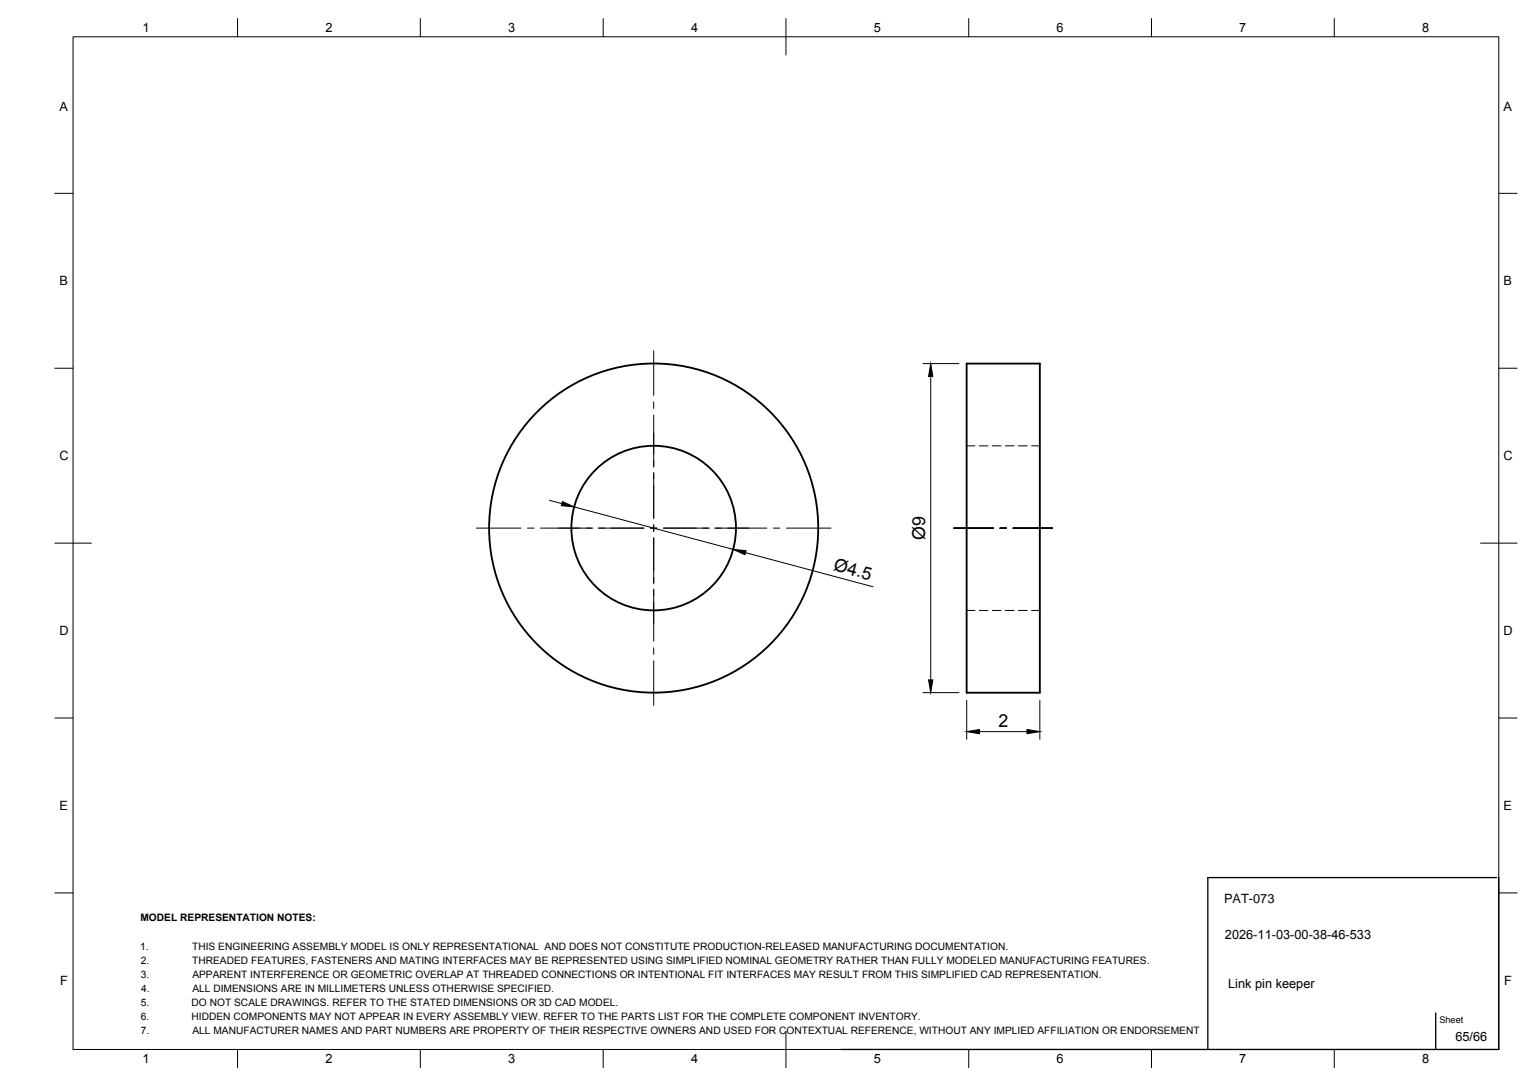
ISO-10303-21;
HEADER;
/* Generated by software containing ST-Developer
 * from STEP Tools, Inc. (www.steptools.com) 
 */

FILE_DESCRIPTION(
/* description */ ('Manual piston pump'),
/* implementation_level */ '2;1');

FILE_NAME(
/* name */ 'Link pin keeper.step',
/* time_stamp */ '2026-11-02T16:54:23-08:00',
/* author */ (''),
/* organization */ (''),
/* preprocessor_version */ 'ST-DEVELOPER v20.2',
/* originating_system */ 'Autodesk Translation Framework v15.17.0.0',
/* authorisation */ '');

FILE_SCHEMA (('AUTOMOTIVE_DESIGN { 1 0 10303 214 3 1 1 }'));
ENDSEC;

DATA;
#10=MECHANICAL_DESIGN_GEOMETRIC_PRESENTATION_REPRESENTATION('',(#757),#19043);
#622=SHAPE_REPRESENTATION_RELATIONSHIP('SRR','None',#19372,#685);
#685=ADVANCED_BREP_SHAPE_REPRESENTATION('',(#825),#19039);
#757=STYLED_ITEM('',(#19661),#825);
#825=MANIFOLD_SOLID_BREP('Body1',#9545);
#1041=FACE_BOUND('',#2631,.T.);
#1042=FACE_BOUND('',#2633,.T.);
#1284=CYLINDRICAL_SURFACE('',#11414,0.225);
#1285=CYLINDRICAL_SURFACE('',#11417,0.449999999999999);
#1839=FACE_OUTER_BOUND('',#2628,.T.);
#1840=FACE_OUTER_BOUND('',#2629,.T.);
#1841=FACE_OUTER_BOUND('',#2630,.T.);
#1842=FACE_OUTER_BOUND('',#2632,.T.);
#2628=EDGE_LOOP('',(#8465,#8466,#8467,#8468));
#2629=EDGE_LOOP('',(#8469,#8470,#8471,#8472));
#2630=EDGE_LOOP('',(#8473));
#2631=EDGE_LOOP('',(#8474));
#2632=EDGE_LOOP('',(#8475));
#2633=EDGE_LOOP('',(#8476));
#3128=CIRCLE('',#11415,0.225);
#3129=CIRCLE('',#11416,0.225);
#3130=CIRCLE('',#11418,0.449999999999999);
#3131=CIRCLE('',#11419,0.449999999999999);
#3716=LINE('',#18755,#4320);
#3717=LINE('',#18761,#4321);
#4320=VECTOR('',#14410,0.225);
#4321=VECTOR('',#14417,0.449999999999999);
#5088=VERTEX_POINT('',#18752);
#5089=VERTEX_POINT('',#18754);
#5090=VERTEX_POINT('',#18758);
#5091=VERTEX_POINT('',#18760);
#6219=EDGE_CURVE('',#5088,#5088,#3128,.T.);
#6220=EDGE_CURVE('',#5088,#5089,#3716,.T.);
#6221=EDGE_CURVE('',#5089,#5089,#3129,.T.);
#6222=EDGE_CURVE('',#5090,#5090,#3130,.T.);
#6223=EDGE_CURVE('',#5090,#5091,#3717,.T.);
#6224=EDGE_CURVE('',#5091,#5091,#3131,.T.);
#8465=ORIENTED_EDGE('',*,*,#6219,.F.);
#8466=ORIENTED_EDGE('',*,*,#6220,.T.);
#8467=ORIENTED_EDGE('',*,*,#6221,.T.);
#8468=ORIENTED_EDGE('',*,*,#6220,.F.);
#8469=ORIENTED_EDGE('',*,*,#6222,.F.);
#8470=ORIENTED_EDGE('',*,*,#6223,.T.);
#8471=ORIENTED_EDGE('',*,*,#6224,.T.);
#8472=ORIENTED_EDGE('',*,*,#6223,.F.);
#8473=ORIENTED_EDGE('',*,*,#6222,.T.);
#8474=ORIENTED_EDGE('',*,*,#6219,.T.);
#8475=ORIENTED_EDGE('',*,*,#6224,.F.);
#8476=ORIENTED_EDGE('',*,*,#6221,.F.);
#8880=PLANE('',#11420);
#8881=PLANE('',#11421);
#9444=ADVANCED_FACE('',(#1839),#1284,.F.);
#9445=ADVANCED_FACE('',(#1840),#1285,.T.);
#9446=ADVANCED_FACE('',(#1841,#1041),#8880,.T.);
#9447=ADVANCED_FACE('',(#1842,#1042),#8881,.F.);
#9545=CLOSED_SHELL('',(#9444,#9445,#9446,#9447));
#11413=AXIS2_PLACEMENT_3D('',#18750,#14404,#14405);
#11414=AXIS2_PLACEMENT_3D('',#18751,#14406,#14407);
#11415=AXIS2_PLACEMENT_3D('',#18753,#14408,#14409);
#11416=AXIS2_PLACEMENT_3D('',#18756,#14411,#14412);
#11417=AXIS2_PLACEMENT_3D('',#18757,#14413,#14414);
#11418=AXIS2_PLACEMENT_3D('',#18759,#14415,#14416);
#11419=AXIS2_PLACEMENT_3D('',#18762,#14418,#14419);
#11420=AXIS2_PLACEMENT_3D('',#18763,#14420,#14421);
#11421=AXIS2_PLACEMENT_3D('',#18764,#14422,#14423);
#14404=DIRECTION('axis',(0.,0.,1.));
#14405=DIRECTION('refdir',(1.,0.,0.));
#14406=DIRECTION('center_axis',(1.,0.,0.));
#14407=DIRECTION('ref_axis',(0.,0.,-1.));
#14408=DIRECTION('center_axis',(-1.,0.,0.));
#14409=DIRECTION('ref_axis',(0.,0.,-1.));
#14410=DIRECTION('',(-1.,0.,0.));
#14411=DIRECTION('center_axis',(-1.,0.,0.));
#14412=DIRECTION('ref_axis',(0.,0.,-1.));
#14413=DIRECTION('center_axis',(1.,0.,0.));
#14414=DIRECTION('ref_axis',(0.,0.,-1.));
#14415=DIRECTION('center_axis',(1.,0.,0.));
#14416=DIRECTION('ref_axis',(0.,0.,-1.));
#14417=DIRECTION('',(-1.,0.,0.));
#14418=DIRECTION('center_axis',(1.,0.,0.));
#14419=DIRECTION('ref_axis',(0.,0.,-1.));
#14420=DIRECTION('center_axis',(1.,0.,0.));
#14421=DIRECTION('ref_axis',(0.,0.,-1.));
#14422=DIRECTION('center_axis',(1.,0.,0.));
#14423=DIRECTION('ref_axis',(0.,0.,-1.));
#18750=CARTESIAN_POINT('',(0.,0.,0.));
#18751=CARTESIAN_POINT('Origin',(0.5,-8.,10.));
#18752=CARTESIAN_POINT('',(0.7,-8.,10.225));
#18753=CARTESIAN_POINT('Origin',(0.7,-8.,10.));
#18754=CARTESIAN_POINT('',(0.5,-8.,10.225));
#18755=CARTESIAN_POINT('',(0.5,-8.,10.225));
#18756=CARTESIAN_POINT('Origin',(0.5,-8.,10.));
#18757=CARTESIAN_POINT('Origin',(0.5,-8.,10.));
#18758=CARTESIAN_POINT('',(0.7,-8.,10.45));
#18759=CARTESIAN_POINT('Origin',(0.7,-8.,10.));
#18760=CARTESIAN_POINT('',(0.5,-8.,10.45));
#18761=CARTESIAN_POINT('',(0.5,-8.,10.45));
#18762=CARTESIAN_POINT('Origin',(0.5,-8.,10.));
#18763=CARTESIAN_POINT('Origin',(0.7,-8.,10.));
#18764=CARTESIAN_POINT('Origin',(0.5,-8.,10.));
#18968=UNCERTAINTY_MEASURE_WITH_UNIT(LENGTH_MEASURE(0.001),#19044,
'DISTANCE_ACCURACY_VALUE',
'Maximum model space distance between geometric entities at asserted c
onnectivities');
#18972=UNCERTAINTY_MEASURE_WITH_UNIT(LENGTH_MEASURE(0.001),#19044,
'DISTANCE_ACCURACY_VALUE',
'Maximum model space distance between geometric entities at asserted c
onnectivities');
#19039=(
GEOMETRIC_REPRESENTATION_CONTEXT(3)
GLOBAL_UNCERTAINTY_ASSIGNED_CONTEXT((#18968))
GLOBAL_UNIT_ASSIGNED_CONTEXT((#19044,#19046,#19047))
REPRESENTATION_CONTEXT('','3D')
);
#19043=(
GEOMETRIC_REPRESENTATION_CONTEXT(3)
GLOBAL_UNCERTAINTY_ASSIGNED_CONTEXT((#18972))
GLOBAL_UNIT_ASSIGNED_CONTEXT((#19044,#19046,#19047))
REPRESENTATION_CONTEXT('','3D')
);
#19044=(
LENGTH_UNIT()
NAMED_UNIT(*)
SI_UNIT(.CENTI.,.METRE.)
);
#19046=(
NAMED_UNIT(*)
PLANE_ANGLE_UNIT()
SI_UNIT($,.RADIAN.)
);
#19047=(
NAMED_UNIT(*)
SI_UNIT($,.STERADIAN.)
SOLID_ANGLE_UNIT()
);
#19114=SHAPE_DEFINITION_REPRESENTATION(#19271,#19372);
#19271=PRODUCT_DEFINITION_SHAPE('',$,#19443);
#19372=SHAPE_REPRESENTATION('',(#11413),#19039);
#19376=PRODUCT_DEFINITION_CONTEXT('part definition',#19588,'design');
#19443=PRODUCT_DEFINITION('2026-11-03-00-38-46-533','Link pin keeper',#19513,
#19376);
#19513=PRODUCT_DEFINITION_FORMATION('',$,#19656);
#19588=APPLICATION_CONTEXT(
'Core Data for Automotive Mechanical Design Process');
#19589=PRODUCT_CONTEXT('part definition',#19588,'mechanical');
#19656=PRODUCT('2026-11-03-00-38-46-533','Link pin keeper',
'Link pin keeper',(#19589));
#19661=PRESENTATION_STYLE_ASSIGNMENT((#19667));
#19667=SURFACE_STYLE_USAGE(.BOTH.,#19673);
#19673=SURFACE_SIDE_STYLE('',(#19679));
#19679=SURFACE_STYLE_FILL_AREA(#19685);
#19685=FILL_AREA_STYLE('CAD Library Painted - Engineering blue',(#19691));
#19691=FILL_AREA_STYLE_COLOUR('CAD Library Painted - Engineering blue',
#19697);
#19697=COLOUR_RGB('CAD Library Painted - Engineering blue',0.12156862745098,
0.356862745098039,0.6);
ENDSEC;
END-ISO-10303-21;
